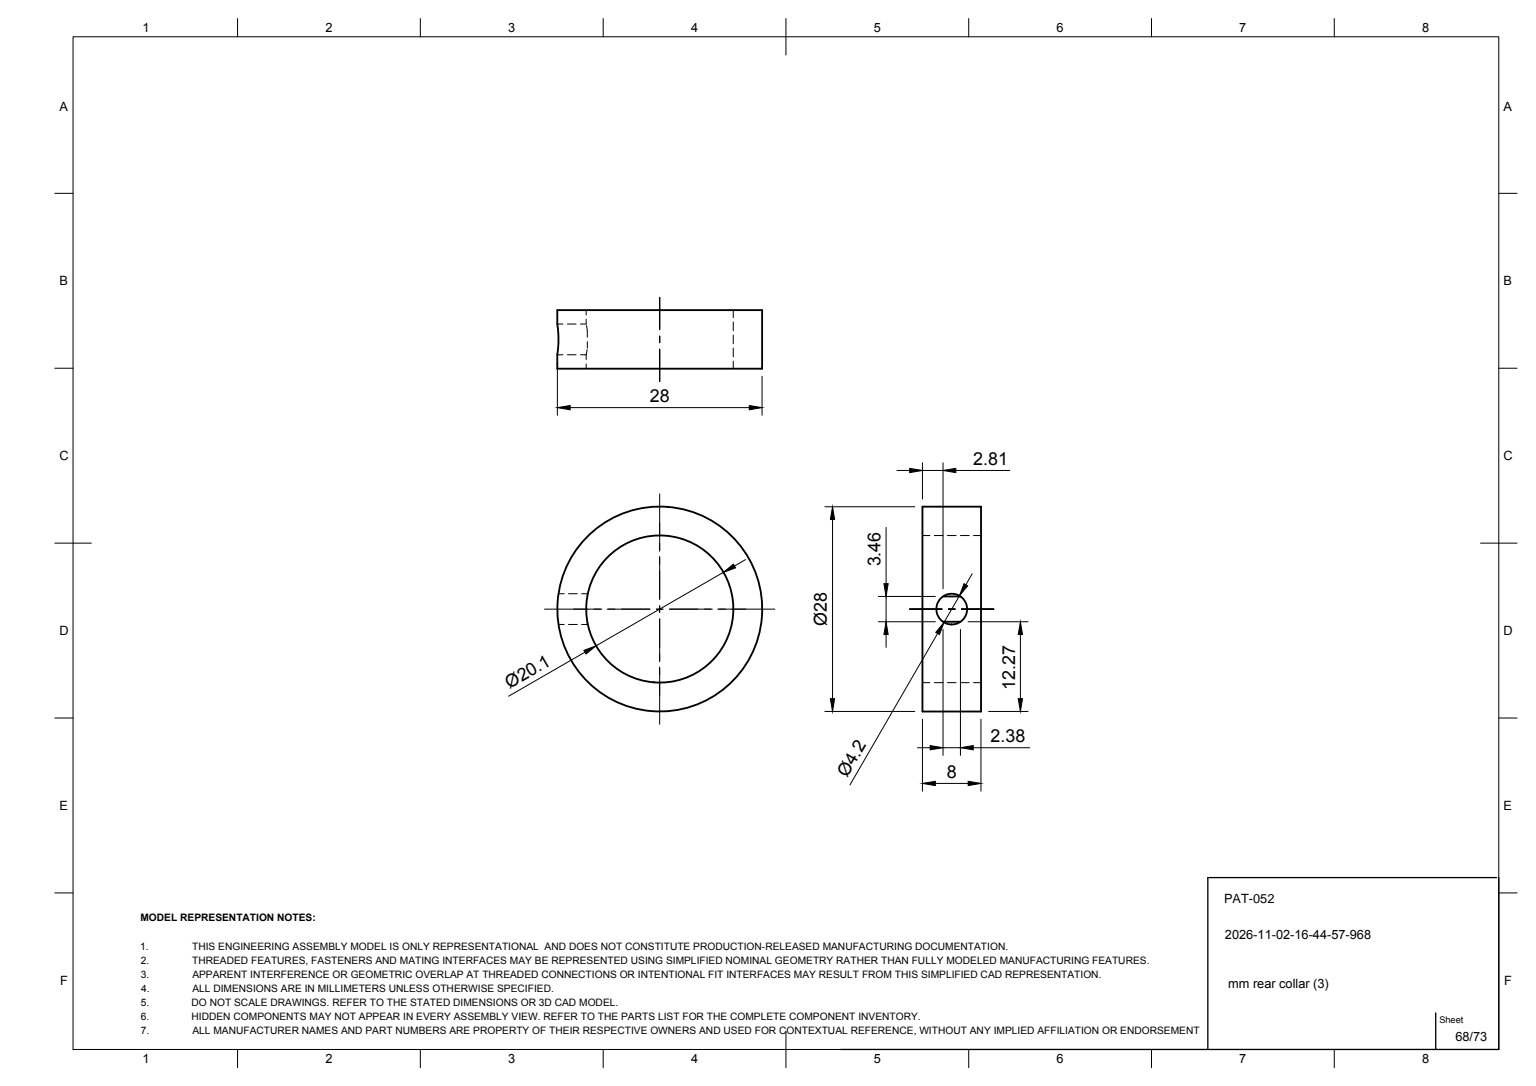
ISO-10303-21;
HEADER;
/* Generated by software containing ST-Developer
 * from STEP Tools, Inc. (www.steptools.com) 
 */

FILE_DESCRIPTION(
/* description */ ('Hand-crank gear train demonstrator'),
/* implementation_level */ '2;1');

FILE_NAME(
/* name */ 'mm rear collar (3).step',
/* time_stamp */ '2026-10-28T03:22:13-07:00',
/* author */ (''),
/* organization */ (''),
/* preprocessor_version */ 'ST-DEVELOPER v20.2',
/* originating_system */ 'Autodesk Translation Framework v15.17.0.0',
/* authorisation */ '');

FILE_SCHEMA (('AUTOMOTIVE_DESIGN { 1 0 10303 214 3 1 1 }'));
ENDSEC;

DATA;
#10=MECHANICAL_DESIGN_GEOMETRIC_PRESENTATION_REPRESENTATION('',(#1258),#62758);
#903=B_SPLINE_CURVE_WITH_KNOTS('',3,(#38516,#38517,#38518,#38519,#38520,
#38521,#38522,#38523,#38524,#38525,#38526,#38527,#38528,#38529),
 .UNSPECIFIED.,.F.,.F.,(4,2,2,2,2,2,4),(0.756005737987044,0.793568827564651,
0.872922520054207,0.952276212543762,1.03162990503332,1.11098359752287,1.14854668710048),
 .UNSPECIFIED.);
#904=B_SPLINE_CURVE_WITH_KNOTS('',3,(#38535,#38536,#38537,#38538,#38539,
#38540,#38541,#38542,#38543,#38544,#38545,#38546,#38547,#38548,#38549,#38550,
#38551,#38552),.UNSPECIFIED.,.F.,.F.,(4,2,2,2,2,2,2,2,4),(0.,0.0792334805614372,
0.158466961122874,0.237699060165218,0.316931159207562,0.396163258249906,
0.47539535729225,0.554628837853687,0.633862318415124),.UNSPECIFIED.);
#905=B_SPLINE_CURVE_WITH_KNOTS('',3,(#38553,#38554,#38555,#38556,#38557,
#38558,#38559,#38560,#38561,#38562,#38563,#38564,#38565,#38566,#38567,#38568,
#38569,#38570),.UNSPECIFIED.,.F.,.F.,(4,2,2,2,2,2,2,2,4),(0.633862318415124,
0.713095798976561,0.792329279537998,0.871561378580342,0.950793477622686,
1.03002557666503,1.10925767570737,1.18849115626881,1.26772463683025),
 .UNSPECIFIED.);
#906=B_SPLINE_CURVE_WITH_KNOTS('',3,(#38573,#38574,#38575,#38576,#38577,
#38578,#38579,#38580,#38581,#38582,#38583,#38584,#38585,#38586),
 .UNSPECIFIED.,.F.,.F.,(4,2,2,2,2,2,4),(0.121154929624534,0.158718019202142,
0.238071711691698,0.317425404181254,0.39677909667081,0.476132789160366,
0.513695878737972),.UNSPECIFIED.);
#1115=SHAPE_REPRESENTATION_RELATIONSHIP('SRR','None',#63093,#1179);
#1179=ADVANCED_BREP_SHAPE_REPRESENTATION('',(#1333),#62747);
#1258=STYLED_ITEM('',(#63448),#1333);
#1333=MANIFOLD_SOLID_BREP('Body1',#16442);
#1611=FACE_BOUND('',#4027,.T.);
#1612=FACE_BOUND('',#4029,.T.);
#1613=FACE_BOUND('',#4031,.T.);
#1614=FACE_BOUND('',#4033,.T.);
#2027=PLANE('',#18420);
#2028=PLANE('',#18425);
#2029=PLANE('',#18432);
#2030=PLANE('',#18433);
#2818=FACE_OUTER_BOUND('',#4023,.T.);
#2819=FACE_OUTER_BOUND('',#4024,.T.);
#2820=FACE_OUTER_BOUND('',#4025,.T.);
#2821=FACE_OUTER_BOUND('',#4026,.T.);
#2822=FACE_OUTER_BOUND('',#4028,.T.);
#2823=FACE_OUTER_BOUND('',#4030,.T.);
#2824=FACE_OUTER_BOUND('',#4032,.T.);
#4023=EDGE_LOOP('',(#13885,#13886));
#4024=EDGE_LOOP('',(#13887,#13888,#13889,#13890,#13891,#13892,#13893,#13894,
#13895));
#4025=EDGE_LOOP('',(#13896,#13897,#13898));
#4026=EDGE_LOOP('',(#13899,#13900,#13901,#13902));
#4027=EDGE_LOOP('',(#13903,#13904,#13905,#13906));
#4028=EDGE_LOOP('',(#13907,#13908,#13909,#13910));
#4029=EDGE_LOOP('',(#13911,#13912));
#4030=EDGE_LOOP('',(#13913));
#4031=EDGE_LOOP('',(#13914));
#4032=EDGE_LOOP('',(#13915));
#4033=EDGE_LOOP('',(#13916));
#5153=LINE('',#38512,#6285);
#5154=LINE('',#38533,#6286);
#5155=LINE('',#38588,#6287);
#5156=LINE('',#38593,#6288);
#5157=LINE('',#38599,#6289);
#6285=VECTOR('',#22224,1.);
#6286=VECTOR('',#22231,0.210000000000001);
#6287=VECTOR('',#22236,1.);
#6288=VECTOR('',#22241,1.005);
#6289=VECTOR('',#22248,1.4);
#7084=CIRCLE('',#18421,0.210000000000001);
#7085=CIRCLE('',#18423,0.210000000000001);
#7086=CIRCLE('',#18424,0.210000000000001);
#7087=CIRCLE('',#18427,1.005);
#7088=CIRCLE('',#18428,1.005);
#7089=CIRCLE('',#18430,1.4);
#7090=CIRCLE('',#18431,1.4);
#8243=VERTEX_POINT('',#38510);
#8244=VERTEX_POINT('',#38511);
#8245=VERTEX_POINT('',#38515);
#8246=VERTEX_POINT('',#38530);
#8247=VERTEX_POINT('',#38532);
#8248=VERTEX_POINT('',#38534);
#8249=VERTEX_POINT('',#38571);
#8250=VERTEX_POINT('',#38590);
#8251=VERTEX_POINT('',#38592);
#8252=VERTEX_POINT('',#38596);
#8253=VERTEX_POINT('',#38598);
#10194=EDGE_CURVE('',#8243,#8244,#5153,.T.);
#10195=EDGE_CURVE('',#8243,#8244,#7084,.T.);
#10196=EDGE_CURVE('',#8245,#8243,#903,.T.);
#10197=EDGE_CURVE('',#8246,#8245,#7085,.T.);
#10198=EDGE_CURVE('',#8246,#8247,#5154,.T.);
#10199=EDGE_CURVE('',#8248,#8247,#904,.T.);
#10200=EDGE_CURVE('',#8247,#8248,#905,.T.);
#10201=EDGE_CURVE('',#8249,#8246,#7086,.T.);
#10202=EDGE_CURVE('',#8244,#8249,#906,.T.);
#10203=EDGE_CURVE('',#8249,#8245,#5155,.T.);
#10204=EDGE_CURVE('',#8250,#8250,#7087,.T.);
#10205=EDGE_CURVE('',#8250,#8251,#5156,.T.);
#10206=EDGE_CURVE('',#8251,#8251,#7088,.T.);
#10207=EDGE_CURVE('',#8252,#8252,#7089,.T.);
#10208=EDGE_CURVE('',#8252,#8253,#5157,.T.);
#10209=EDGE_CURVE('',#8253,#8253,#7090,.T.);
#13885=ORIENTED_EDGE('',*,*,#10194,.F.);
#13886=ORIENTED_EDGE('',*,*,#10195,.T.);
#13887=ORIENTED_EDGE('',*,*,#10196,.F.);
#13888=ORIENTED_EDGE('',*,*,#10197,.F.);
#13889=ORIENTED_EDGE('',*,*,#10198,.T.);
#13890=ORIENTED_EDGE('',*,*,#10199,.F.);
#13891=ORIENTED_EDGE('',*,*,#10200,.F.);
#13892=ORIENTED_EDGE('',*,*,#10198,.F.);
#13893=ORIENTED_EDGE('',*,*,#10201,.F.);
#13894=ORIENTED_EDGE('',*,*,#10202,.F.);
#13895=ORIENTED_EDGE('',*,*,#10195,.F.);
#13896=ORIENTED_EDGE('',*,*,#10203,.F.);
#13897=ORIENTED_EDGE('',*,*,#10201,.T.);
#13898=ORIENTED_EDGE('',*,*,#10197,.T.);
#13899=ORIENTED_EDGE('',*,*,#10204,.F.);
#13900=ORIENTED_EDGE('',*,*,#10205,.T.);
#13901=ORIENTED_EDGE('',*,*,#10206,.T.);
#13902=ORIENTED_EDGE('',*,*,#10205,.F.);
#13903=ORIENTED_EDGE('',*,*,#10202,.T.);
#13904=ORIENTED_EDGE('',*,*,#10203,.T.);
#13905=ORIENTED_EDGE('',*,*,#10196,.T.);
#13906=ORIENTED_EDGE('',*,*,#10194,.T.);
#13907=ORIENTED_EDGE('',*,*,#10207,.F.);
#13908=ORIENTED_EDGE('',*,*,#10208,.T.);
#13909=ORIENTED_EDGE('',*,*,#10209,.T.);
#13910=ORIENTED_EDGE('',*,*,#10208,.F.);
#13911=ORIENTED_EDGE('',*,*,#10199,.T.);
#13912=ORIENTED_EDGE('',*,*,#10200,.T.);
#13913=ORIENTED_EDGE('',*,*,#10207,.T.);
#13914=ORIENTED_EDGE('',*,*,#10204,.T.);
#13915=ORIENTED_EDGE('',*,*,#10209,.F.);
#13916=ORIENTED_EDGE('',*,*,#10206,.F.);
#15374=CYLINDRICAL_SURFACE('',#18422,0.210000000000001);
#15375=CYLINDRICAL_SURFACE('',#18426,1.005);
#15376=CYLINDRICAL_SURFACE('',#18429,1.4);
#16128=ADVANCED_FACE('',(#2818),#2027,.T.);
#16129=ADVANCED_FACE('',(#2819),#15374,.F.);
#16130=ADVANCED_FACE('',(#2820),#2028,.T.);
#16131=ADVANCED_FACE('',(#2821,#1611),#15375,.F.);
#16132=ADVANCED_FACE('',(#2822,#1612),#15376,.T.);
#16133=ADVANCED_FACE('',(#2823,#1613),#2029,.T.);
#16134=ADVANCED_FACE('',(#2824,#1614),#2030,.F.);
#16442=CLOSED_SHELL('',(#16128,#16129,#16130,#16131,#16132,#16133,#16134));
#18419=AXIS2_PLACEMENT_3D('',#38508,#22220,#22221);
#18420=AXIS2_PLACEMENT_3D('',#38509,#22222,#22223);
#18421=AXIS2_PLACEMENT_3D('',#38513,#22225,#22226);
#18422=AXIS2_PLACEMENT_3D('',#38514,#22227,#22228);
#18423=AXIS2_PLACEMENT_3D('',#38531,#22229,#22230);
#18424=AXIS2_PLACEMENT_3D('',#38572,#22232,#22233);
#18425=AXIS2_PLACEMENT_3D('',#38587,#22234,#22235);
#18426=AXIS2_PLACEMENT_3D('',#38589,#22237,#22238);
#18427=AXIS2_PLACEMENT_3D('',#38591,#22239,#22240);
#18428=AXIS2_PLACEMENT_3D('',#38594,#22242,#22243);
#18429=AXIS2_PLACEMENT_3D('',#38595,#22244,#22245);
#18430=AXIS2_PLACEMENT_3D('',#38597,#22246,#22247);
#18431=AXIS2_PLACEMENT_3D('',#38600,#22249,#22250);
#18432=AXIS2_PLACEMENT_3D('',#38601,#22251,#22252);
#18433=AXIS2_PLACEMENT_3D('',#38602,#22253,#22254);
#22220=DIRECTION('axis',(0.,0.,1.));
#22221=DIRECTION('refdir',(1.,0.,0.));
#22222=DIRECTION('center_axis',(0.,0.,1.));
#22223=DIRECTION('ref_axis',(1.,0.,0.));
#22224=DIRECTION('',(0.,1.,0.));
#22225=DIRECTION('center_axis',(0.,0.,1.));
#22226=DIRECTION('ref_axis',(1.,0.,0.));
#22227=DIRECTION('center_axis',(0.,0.,1.));
#22228=DIRECTION('ref_axis',(1.,0.,0.));
#22229=DIRECTION('center_axis',(0.,0.,1.));
#22230=DIRECTION('ref_axis',(1.,0.,0.));
#22231=DIRECTION('',(0.,0.,1.));
#22232=DIRECTION('center_axis',(0.,0.,1.));
#22233=DIRECTION('ref_axis',(1.,0.,0.));
#22234=DIRECTION('center_axis',(0.,0.,1.));
#22235=DIRECTION('ref_axis',(1.,0.,0.));
#22236=DIRECTION('',(0.,-1.,0.));
#22237=DIRECTION('center_axis',(0.,1.,0.));
#22238=DIRECTION('ref_axis',(1.,0.,0.));
#22239=DIRECTION('center_axis',(0.,-1.,0.));
#22240=DIRECTION('ref_axis',(1.,0.,0.));
#22241=DIRECTION('',(0.,-1.,0.));
#22242=DIRECTION('center_axis',(0.,-1.,0.));
#22243=DIRECTION('ref_axis',(1.,0.,0.));
#22244=DIRECTION('center_axis',(0.,1.,0.));
#22245=DIRECTION('ref_axis',(1.,0.,0.));
#22246=DIRECTION('center_axis',(0.,1.,0.));
#22247=DIRECTION('ref_axis',(1.,0.,0.));
#22248=DIRECTION('',(0.,-1.,0.));
#22249=DIRECTION('center_axis',(0.,1.,0.));
#22250=DIRECTION('ref_axis',(1.,0.,0.));
#22251=DIRECTION('center_axis',(0.,1.,0.));
#22252=DIRECTION('ref_axis',(1.,0.,0.));
#22253=DIRECTION('center_axis',(0.,1.,0.));
#22254=DIRECTION('ref_axis',(1.,0.,0.));
#38508=CARTESIAN_POINT('',(0.,0.,0.));
#38509=CARTESIAN_POINT('Origin',(18.,-3.2,9.99));
#38510=CARTESIAN_POINT('',(18.17298843892,-3.31905880899793,9.99));
#38511=CARTESIAN_POINT('',(18.17298843892,-3.08094119100207,9.99));
#38512=CARTESIAN_POINT('',(18.17298843892,-3.6,9.99));
#38513=CARTESIAN_POINT('Origin',(18.,-3.2,9.99));
#38514=CARTESIAN_POINT('Origin',(18.,-3.2,9.99));
#38515=CARTESIAN_POINT('',(17.82701156108,-3.31905880899793,9.99));
#38516=CARTESIAN_POINT('Ctrl Pts',(17.82701156108,-3.31905880899793,9.99));
#38517=CARTESIAN_POINT('Ctrl Pts',(17.8344051346887,-3.3298014223953,9.99129192197638));
#38518=CARTESIAN_POINT('Ctrl Pts',(17.8427028612744,-3.33968770937275,9.99265394943905));
#38519=CARTESIAN_POINT('Ctrl Pts',(17.8701079261549,-3.36709277425327,9.9967480843909));
#38520=CARTESIAN_POINT('Ctrl Pts',(17.8936698322407,-3.38324205633295,9.99969589327638));
#38521=CARTESIAN_POINT('Ctrl Pts',(17.9453870953676,-3.40469779396491,10.0038502947236));
#38522=CARTESIAN_POINT('Ctrl Pts',(17.9735487691701,-3.41,10.005));
#38523=CARTESIAN_POINT('Ctrl Pts',(18.0264512308299,-3.41,10.005));
#38524=CARTESIAN_POINT('Ctrl Pts',(18.0546129046324,-3.40469779396491,10.0038502947236));
#38525=CARTESIAN_POINT('Ctrl Pts',(18.1063301677593,-3.38324205633295,9.99969589327638));
#38526=CARTESIAN_POINT('Ctrl Pts',(18.1298920738451,-3.36709277425327,9.9967480843909));
#38527=CARTESIAN_POINT('Ctrl Pts',(18.1572971387256,-3.33968770937275,9.99265394943905));
#38528=CARTESIAN_POINT('Ctrl Pts',(18.1655948653113,-3.3298014223953,9.99129192197638));
#38529=CARTESIAN_POINT('Ctrl Pts',(18.17298843892,-3.31905880899793,9.99));
#38530=CARTESIAN_POINT('',(17.79,-3.2,9.99));
#38531=CARTESIAN_POINT('Origin',(18.,-3.2,9.99));
#38532=CARTESIAN_POINT('',(17.79,-3.2,10.38416039533));
#38533=CARTESIAN_POINT('',(17.79,-3.2,9.99));
#38534=CARTESIAN_POINT('',(18.21,-3.2,10.38416039533));
#38535=CARTESIAN_POINT('Ctrl Pts',(18.21,-3.2,10.38416039533));
#38536=CARTESIAN_POINT('Ctrl Pts',(18.21,-3.22641116018715,10.38416039533));
#38537=CARTESIAN_POINT('Ctrl Pts',(18.2047135491119,-3.2545550596171,10.3849944296993));
#38538=CARTESIAN_POINT('Ctrl Pts',(18.1832699958585,-3.30628264999174,10.3879947099895));
#38539=CARTESIAN_POINT('Ctrl Pts',(18.1671150376064,-3.32986981049193,10.3901162943626));
#38540=CARTESIAN_POINT('Ctrl Pts',(18.1298701351968,-3.36711471290157,10.394089123191));
#38541=CARTESIAN_POINT('Ctrl Pts',(18.1062828345902,-3.38326992585508,10.3962002442067));
#38542=CARTESIAN_POINT('Ctrl Pts',(18.0545547656039,-3.40471366447292,10.3991765222353));
#38543=CARTESIAN_POINT('Ctrl Pts',(18.0264106996808,-3.41,10.4));
#38544=CARTESIAN_POINT('Ctrl Pts',(17.9735893003192,-3.41,10.4));
#38545=CARTESIAN_POINT('Ctrl Pts',(17.9454452343961,-3.40471366447292,10.3991765222353));
#38546=CARTESIAN_POINT('Ctrl Pts',(17.8937171654098,-3.38326992585508,10.3962002442067));
#38547=CARTESIAN_POINT('Ctrl Pts',(17.8701298648032,-3.36711471290157,10.394089123191));
#38548=CARTESIAN_POINT('Ctrl Pts',(17.8328849623936,-3.32986981049193,10.3901162943626));
#38549=CARTESIAN_POINT('Ctrl Pts',(17.8167300041415,-3.30628264999174,10.3879947099895));
#38550=CARTESIAN_POINT('Ctrl Pts',(17.7952864508881,-3.2545550596171,10.3849944296993));
#38551=CARTESIAN_POINT('Ctrl Pts',(17.79,-3.22641116018715,10.38416039533));
#38552=CARTESIAN_POINT('Ctrl Pts',(17.79,-3.2,10.38416039533));
#38553=CARTESIAN_POINT('Ctrl Pts',(17.79,-3.2,10.38416039533));
#38554=CARTESIAN_POINT('Ctrl Pts',(17.79,-3.17358883981285,10.38416039533));
#38555=CARTESIAN_POINT('Ctrl Pts',(17.7952864508881,-3.1454449403829,10.3849944296993));
#38556=CARTESIAN_POINT('Ctrl Pts',(17.8167300041415,-3.09371735000826,10.3879947099895));
#38557=CARTESIAN_POINT('Ctrl Pts',(17.8328849623936,-3.07013018950808,10.3901162943626));
#38558=CARTESIAN_POINT('Ctrl Pts',(17.8701298648032,-3.03288528709843,10.394089123191));
#38559=CARTESIAN_POINT('Ctrl Pts',(17.8937171654098,-3.01673007414492,10.3962002442067));
#38560=CARTESIAN_POINT('Ctrl Pts',(17.9454452343961,-2.99528633552708,10.3991765222353));
#38561=CARTESIAN_POINT('Ctrl Pts',(17.9735893003192,-2.99,10.4));
#38562=CARTESIAN_POINT('Ctrl Pts',(18.0264106996808,-2.99,10.4));
#38563=CARTESIAN_POINT('Ctrl Pts',(18.0545547656039,-2.99528633552708,10.3991765222353));
#38564=CARTESIAN_POINT('Ctrl Pts',(18.1062828345902,-3.01673007414492,10.3962002442067));
#38565=CARTESIAN_POINT('Ctrl Pts',(18.1298701351968,-3.03288528709843,10.394089123191));
#38566=CARTESIAN_POINT('Ctrl Pts',(18.1671150376064,-3.07013018950807,10.3901162943626));
#38567=CARTESIAN_POINT('Ctrl Pts',(18.1832699958585,-3.09371735000826,10.3879947099895));
#38568=CARTESIAN_POINT('Ctrl Pts',(18.2047135491119,-3.1454449403829,10.3849944296993));
#38569=CARTESIAN_POINT('Ctrl Pts',(18.21,-3.17358883981285,10.38416039533));
#38570=CARTESIAN_POINT('Ctrl Pts',(18.21,-3.2,10.38416039533));
#38571=CARTESIAN_POINT('',(17.82701156108,-3.08094119100207,9.99));
#38572=CARTESIAN_POINT('Origin',(18.,-3.2,9.99));
#38573=CARTESIAN_POINT('Ctrl Pts',(18.17298843892,-3.08094119100207,9.99));
#38574=CARTESIAN_POINT('Ctrl Pts',(18.1655948653113,-3.0701985776047,9.99129192197638));
#38575=CARTESIAN_POINT('Ctrl Pts',(18.1572971387256,-3.06031229062725,9.99265394943905));
#38576=CARTESIAN_POINT('Ctrl Pts',(18.1298920738451,-3.03290722574673,9.9967480843909));
#38577=CARTESIAN_POINT('Ctrl Pts',(18.1063301677593,-3.01675794366705,9.99969589327638));
#38578=CARTESIAN_POINT('Ctrl Pts',(18.0546129046324,-2.99530220603509,10.0038502947236));
#38579=CARTESIAN_POINT('Ctrl Pts',(18.0264512308299,-2.99,10.005));
#38580=CARTESIAN_POINT('Ctrl Pts',(17.9735487691701,-2.99,10.005));
#38581=CARTESIAN_POINT('Ctrl Pts',(17.9453870953676,-2.99530220603509,10.0038502947236));
#38582=CARTESIAN_POINT('Ctrl Pts',(17.8936698322407,-3.01675794366705,9.99969589327638));
#38583=CARTESIAN_POINT('Ctrl Pts',(17.8701079261549,-3.03290722574673,9.9967480843909));
#38584=CARTESIAN_POINT('Ctrl Pts',(17.8427028612744,-3.06031229062725,9.99265394943905));
#38585=CARTESIAN_POINT('Ctrl Pts',(17.8344051346887,-3.0701985776047,9.99129192197638));
#38586=CARTESIAN_POINT('Ctrl Pts',(17.82701156108,-3.08094119100207,9.99));
#38587=CARTESIAN_POINT('Origin',(18.,-3.2,9.99));
#38588=CARTESIAN_POINT('',(17.82701156108,-3.6,9.99));
#38589=CARTESIAN_POINT('Origin',(18.,-3.6,9.));
#38590=CARTESIAN_POINT('',(16.995,-2.8,9.));
#38591=CARTESIAN_POINT('Origin',(18.,-2.8,9.));
#38592=CARTESIAN_POINT('',(16.995,-3.6,9.));
#38593=CARTESIAN_POINT('',(16.995,-3.6,9.));
#38594=CARTESIAN_POINT('Origin',(18.,-3.6,9.));
#38595=CARTESIAN_POINT('Origin',(18.,-3.6,9.));
#38596=CARTESIAN_POINT('',(16.6,-2.8,9.));
#38597=CARTESIAN_POINT('Origin',(18.,-2.8,9.));
#38598=CARTESIAN_POINT('',(16.6,-3.6,9.));
#38599=CARTESIAN_POINT('',(16.6,-3.6,9.));
#38600=CARTESIAN_POINT('Origin',(18.,-3.6,9.));
#38601=CARTESIAN_POINT('Origin',(18.,-2.8,9.));
#38602=CARTESIAN_POINT('Origin',(18.,-3.6,9.));
#62673=UNCERTAINTY_MEASURE_WITH_UNIT(LENGTH_MEASURE(0.001),#62759,
'DISTANCE_ACCURACY_VALUE',
'Maximum model space distance between geometric entities at asserted c
onnectivities');
#62684=UNCERTAINTY_MEASURE_WITH_UNIT(LENGTH_MEASURE(0.001),#62759,
'DISTANCE_ACCURACY_VALUE',
'Maximum model space distance between geometric entities at asserted c
onnectivities');
#62747=(
GEOMETRIC_REPRESENTATION_CONTEXT(3)
GLOBAL_UNCERTAINTY_ASSIGNED_CONTEXT((#62673))
GLOBAL_UNIT_ASSIGNED_CONTEXT((#62759,#62761,#62762))
REPRESENTATION_CONTEXT('','3D')
);
#62758=(
GEOMETRIC_REPRESENTATION_CONTEXT(3)
GLOBAL_UNCERTAINTY_ASSIGNED_CONTEXT((#62684))
GLOBAL_UNIT_ASSIGNED_CONTEXT((#62759,#62761,#62762))
REPRESENTATION_CONTEXT('','3D')
);
#62759=(
LENGTH_UNIT()
NAMED_UNIT(*)
SI_UNIT(.CENTI.,.METRE.)
);
#62761=(
NAMED_UNIT(*)
PLANE_ANGLE_UNIT()
SI_UNIT($,.RADIAN.)
);
#62762=(
NAMED_UNIT(*)
SI_UNIT($,.STERADIAN.)
SOLID_ANGLE_UNIT()
);
#62825=SHAPE_DEFINITION_REPRESENTATION(#62908,#63093);
#62908=PRODUCT_DEFINITION_SHAPE('',$,#63167);
#63093=SHAPE_REPRESENTATION('',(#18419),#62747);
#63104=PRODUCT_DEFINITION_CONTEXT('part definition',#63325,'design');
#63167=PRODUCT_DEFINITION('mm rear collar (3)','mm rear collar (3)',#63240,
#63104);
#63240=PRODUCT_DEFINITION_FORMATION('',$,#63389);
#63325=APPLICATION_CONTEXT(
'Core Data for Automotive Mechanical Design Process');
#63326=PRODUCT_CONTEXT('part definition',#63325,'mechanical');
#63389=PRODUCT('mm rear collar (3)','mm rear collar (3)','mm rear collar (3)',
(#63326));
#63442=COLOUR_RGB('Light Blue',0.38,0.62,0.78);
#63443=FILL_AREA_STYLE_COLOUR('',#63442);
#63444=FILL_AREA_STYLE('',(#63443));
#63445=SURFACE_STYLE_FILL_AREA(#63444);
#63446=SURFACE_SIDE_STYLE('',(#63445));
#63447=SURFACE_STYLE_USAGE(.BOTH.,#63446);
#63448=PRESENTATION_STYLE_ASSIGNMENT((#63447));
ENDSEC;
END-ISO-10303-21;
